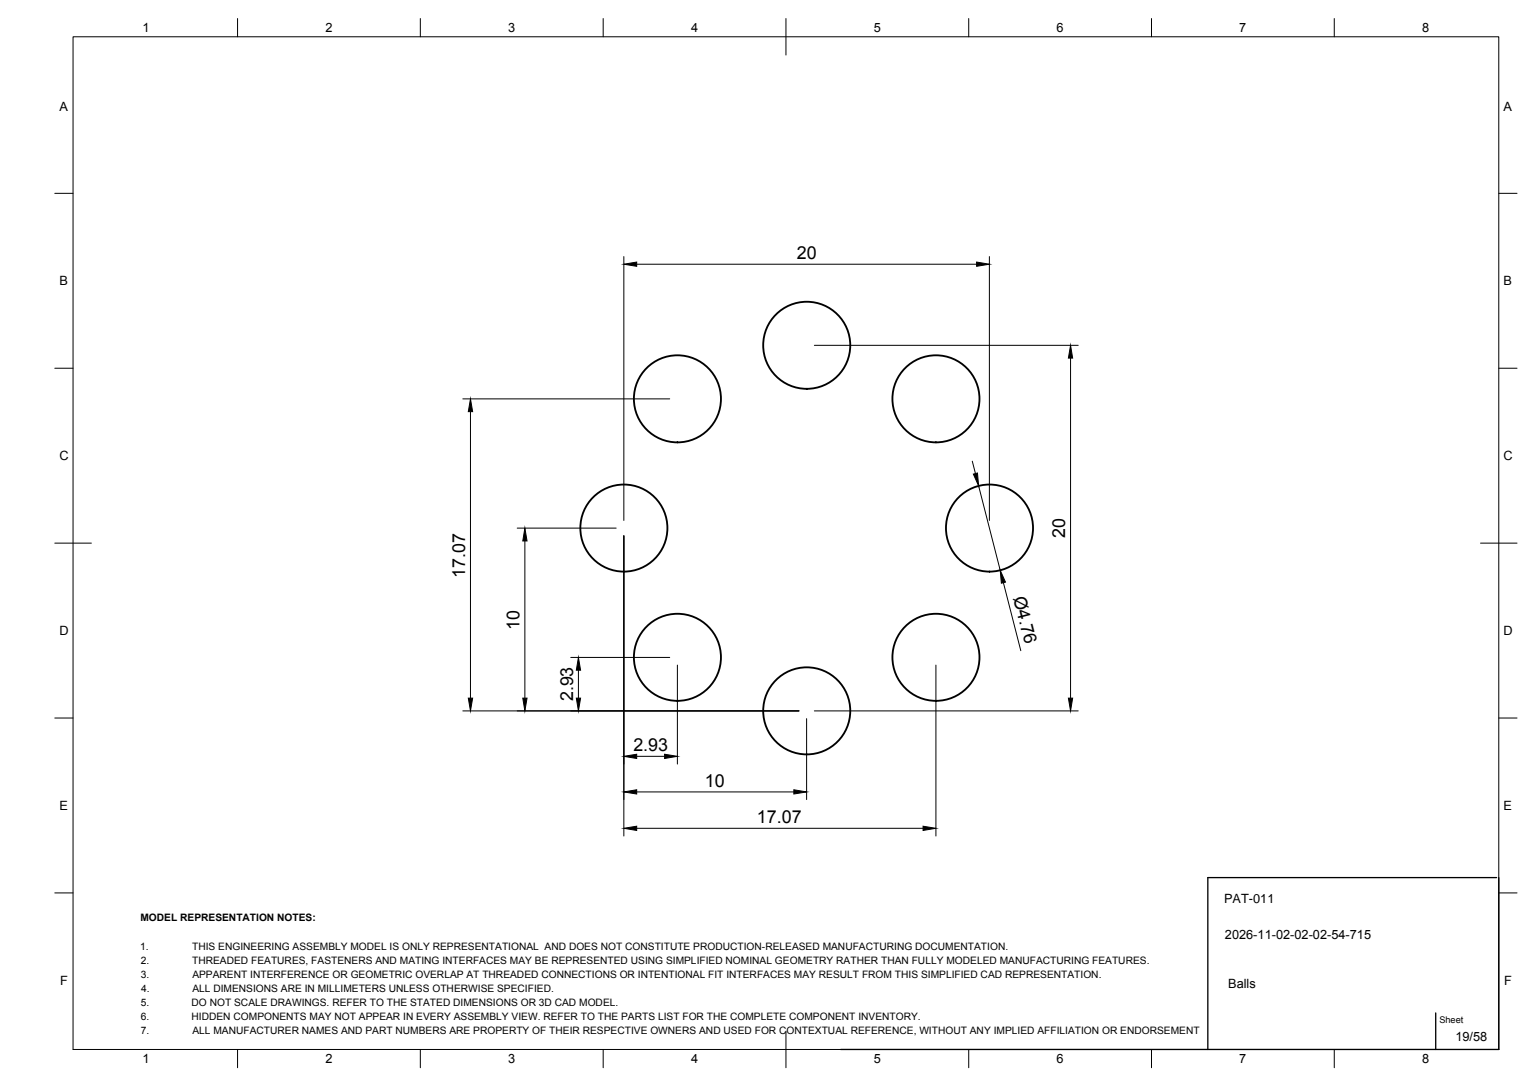
ISO-10303-21;
HEADER;
/* Generated by software containing ST-Developer
 * from STEP Tools, Inc. (www.steptools.com) 
 */

FILE_DESCRIPTION(
/* description */ ('Belt tension measurement rig'),
/* implementation_level */ '2;1');

FILE_NAME(
/* name */ 'Balls.step',
/* time_stamp */ '2026-10-28T03:24:44-07:00',
/* author */ (''),
/* organization */ (''),
/* preprocessor_version */ 'ST-DEVELOPER v20.2',
/* originating_system */ 'Autodesk Translation Framework v15.17.0.0',
/* authorisation */ '');

FILE_SCHEMA (('AUTOMOTIVE_DESIGN { 1 0 10303 214 3 1 1 }'));
ENDSEC;

DATA;
#10=MECHANICAL_DESIGN_GEOMETRIC_PRESENTATION_REPRESENTATION('',(#708,#709,#710,#711,#712,#713,#714,#715),#23587);
#437=SPHERICAL_SURFACE('',#13263,0.23815);
#438=SPHERICAL_SURFACE('',#13265,0.23815);
#439=SPHERICAL_SURFACE('',#13267,0.23815);
#440=SPHERICAL_SURFACE('',#13269,0.23815);
#441=SPHERICAL_SURFACE('',#13271,0.23815);
#442=SPHERICAL_SURFACE('',#13273,0.23815);
#443=SPHERICAL_SURFACE('',#13275,0.23815);
#444=SPHERICAL_SURFACE('',#13277,0.23815);
#598=SHAPE_REPRESENTATION_RELATIONSHIP('SRR','None',#23844,#653);
#653=ADVANCED_BREP_SHAPE_REPRESENTATION('',(#778,#779,#780,#781,#782,#783,
#784,#785),#23542);
#708=STYLED_ITEM('',(#24211),#778);
#709=STYLED_ITEM('',(#24211),#779);
#710=STYLED_ITEM('',(#24211),#780);
#711=STYLED_ITEM('',(#24211),#781);
#712=STYLED_ITEM('',(#24211),#782);
#713=STYLED_ITEM('',(#24211),#783);
#714=STYLED_ITEM('',(#24211),#784);
#715=STYLED_ITEM('',(#24211),#785);
#778=MANIFOLD_SOLID_BREP('Body1',#12213);
#779=MANIFOLD_SOLID_BREP('Body2',#12214);
#780=MANIFOLD_SOLID_BREP('Body3',#12215);
#781=MANIFOLD_SOLID_BREP('Body4',#12216);
#782=MANIFOLD_SOLID_BREP('Body5',#12217);
#783=MANIFOLD_SOLID_BREP('Body6',#12218);
#784=MANIFOLD_SOLID_BREP('Body7',#12219);
#785=MANIFOLD_SOLID_BREP('Body8',#12220);
#1545=FACE_OUTER_BOUND('',#2331,.T.);
#1546=FACE_OUTER_BOUND('',#2332,.T.);
#1547=FACE_OUTER_BOUND('',#2333,.T.);
#1548=FACE_OUTER_BOUND('',#2334,.T.);
#1549=FACE_OUTER_BOUND('',#2335,.T.);
#1550=FACE_OUTER_BOUND('',#2336,.T.);
#1551=FACE_OUTER_BOUND('',#2337,.T.);
#1552=FACE_OUTER_BOUND('',#2338,.T.);
#2331=EDGE_LOOP('',(#8748,#8749));
#2332=EDGE_LOOP('',(#8750,#8751));
#2333=EDGE_LOOP('',(#8752,#8753));
#2334=EDGE_LOOP('',(#8754,#8755));
#2335=EDGE_LOOP('',(#8756,#8757));
#2336=EDGE_LOOP('',(#8758,#8759));
#2337=EDGE_LOOP('',(#8760,#8761));
#2338=EDGE_LOOP('',(#8762,#8763));
#4644=CIRCLE('',#13264,0.23815);
#4645=CIRCLE('',#13266,0.23815);
#4646=CIRCLE('',#13268,0.23815);
#4647=CIRCLE('',#13270,0.23815);
#4648=CIRCLE('',#13272,0.23815);
#4649=CIRCLE('',#13274,0.23815);
#4650=CIRCLE('',#13276,0.23815);
#4651=CIRCLE('',#13278,0.23815);
#5504=VERTEX_POINT('',#19507);
#5505=VERTEX_POINT('',#19508);
#5506=VERTEX_POINT('',#19511);
#5507=VERTEX_POINT('',#19512);
#5508=VERTEX_POINT('',#19515);
#5509=VERTEX_POINT('',#19516);
#5510=VERTEX_POINT('',#19519);
#5511=VERTEX_POINT('',#19520);
#5512=VERTEX_POINT('',#19523);
#5513=VERTEX_POINT('',#19524);
#5514=VERTEX_POINT('',#19527);
#5515=VERTEX_POINT('',#19528);
#5516=VERTEX_POINT('',#19531);
#5517=VERTEX_POINT('',#19532);
#5518=VERTEX_POINT('',#19535);
#5519=VERTEX_POINT('',#19536);
#6733=EDGE_CURVE('',#5504,#5505,#4644,.T.);
#6734=EDGE_CURVE('',#5506,#5507,#4645,.T.);
#6735=EDGE_CURVE('',#5508,#5509,#4646,.T.);
#6736=EDGE_CURVE('',#5510,#5511,#4647,.T.);
#6737=EDGE_CURVE('',#5512,#5513,#4648,.T.);
#6738=EDGE_CURVE('',#5514,#5515,#4649,.T.);
#6739=EDGE_CURVE('',#5516,#5517,#4650,.T.);
#6740=EDGE_CURVE('',#5518,#5519,#4651,.T.);
#8748=ORIENTED_EDGE('',*,*,#6733,.T.);
#8749=ORIENTED_EDGE('',*,*,#6733,.F.);
#8750=ORIENTED_EDGE('',*,*,#6734,.T.);
#8751=ORIENTED_EDGE('',*,*,#6734,.F.);
#8752=ORIENTED_EDGE('',*,*,#6735,.T.);
#8753=ORIENTED_EDGE('',*,*,#6735,.F.);
#8754=ORIENTED_EDGE('',*,*,#6736,.T.);
#8755=ORIENTED_EDGE('',*,*,#6736,.F.);
#8756=ORIENTED_EDGE('',*,*,#6737,.T.);
#8757=ORIENTED_EDGE('',*,*,#6737,.F.);
#8758=ORIENTED_EDGE('',*,*,#6738,.T.);
#8759=ORIENTED_EDGE('',*,*,#6738,.F.);
#8760=ORIENTED_EDGE('',*,*,#6739,.T.);
#8761=ORIENTED_EDGE('',*,*,#6739,.F.);
#8762=ORIENTED_EDGE('',*,*,#6740,.T.);
#8763=ORIENTED_EDGE('',*,*,#6740,.F.);
#11686=ADVANCED_FACE('',(#1545),#437,.T.);
#11687=ADVANCED_FACE('',(#1546),#438,.T.);
#11688=ADVANCED_FACE('',(#1547),#439,.T.);
#11689=ADVANCED_FACE('',(#1548),#440,.T.);
#11690=ADVANCED_FACE('',(#1549),#441,.T.);
#11691=ADVANCED_FACE('',(#1550),#442,.T.);
#11692=ADVANCED_FACE('',(#1551),#443,.T.);
#11693=ADVANCED_FACE('',(#1552),#444,.T.);
#12213=CLOSED_SHELL('',(#11686));
#12214=CLOSED_SHELL('',(#11687));
#12215=CLOSED_SHELL('',(#11688));
#12216=CLOSED_SHELL('',(#11689));
#12217=CLOSED_SHELL('',(#11690));
#12218=CLOSED_SHELL('',(#11691));
#12219=CLOSED_SHELL('',(#11692));
#12220=CLOSED_SHELL('',(#11693));
#13262=AXIS2_PLACEMENT_3D('',#19505,#15516,#15517);
#13263=AXIS2_PLACEMENT_3D('',#19506,#15518,#15519);
#13264=AXIS2_PLACEMENT_3D('',#19509,#15520,#15521);
#13265=AXIS2_PLACEMENT_3D('',#19510,#15522,#15523);
#13266=AXIS2_PLACEMENT_3D('',#19513,#15524,#15525);
#13267=AXIS2_PLACEMENT_3D('',#19514,#15526,#15527);
#13268=AXIS2_PLACEMENT_3D('',#19517,#15528,#15529);
#13269=AXIS2_PLACEMENT_3D('',#19518,#15530,#15531);
#13270=AXIS2_PLACEMENT_3D('',#19521,#15532,#15533);
#13271=AXIS2_PLACEMENT_3D('',#19522,#15534,#15535);
#13272=AXIS2_PLACEMENT_3D('',#19525,#15536,#15537);
#13273=AXIS2_PLACEMENT_3D('',#19526,#15538,#15539);
#13274=AXIS2_PLACEMENT_3D('',#19529,#15540,#15541);
#13275=AXIS2_PLACEMENT_3D('',#19530,#15542,#15543);
#13276=AXIS2_PLACEMENT_3D('',#19533,#15544,#15545);
#13277=AXIS2_PLACEMENT_3D('',#19534,#15546,#15547);
#13278=AXIS2_PLACEMENT_3D('',#19537,#15548,#15549);
#15516=DIRECTION('axis',(0.,0.,1.));
#15517=DIRECTION('refdir',(1.,0.,0.));
#15518=DIRECTION('center_axis',(0.,0.,1.));
#15519=DIRECTION('ref_axis',(1.,0.,0.));
#15520=DIRECTION('center_axis',(1.22464679914735E-16,-1.,0.));
#15521=DIRECTION('ref_axis',(-1.,-1.22464679914735E-16,0.));
#15522=DIRECTION('center_axis',(0.707106781186548,0.,0.707106781186548));
#15523=DIRECTION('ref_axis',(0.707106781186548,0.,-0.707106781186548));
#15524=DIRECTION('center_axis',(8.65956056235494E-17,-1.,-8.65956056235493E-17));
#15525=DIRECTION('ref_axis',(-0.707106781186547,-1.22464679914735E-16,0.707106781186547));
#15526=DIRECTION('center_axis',(1.,0.,0.));
#15527=DIRECTION('ref_axis',(6.12323399573676E-17,0.,-1.));
#15528=DIRECTION('center_axis',(7.49879891330929E-33,-1.,-1.22464679914735E-16));
#15529=DIRECTION('ref_axis',(-6.12323399573676E-17,-1.22464679914735E-16,
1.));
#15530=DIRECTION('center_axis',(0.707106781186548,0.,-0.707106781186548));
#15531=DIRECTION('ref_axis',(-0.707106781186548,0.,-0.707106781186548));
#15532=DIRECTION('center_axis',(-8.65956056235493E-17,-1.,-8.65956056235494E-17));
#15533=DIRECTION('ref_axis',(0.707106781186547,-1.22464679914735E-16,0.707106781186547));
#15534=DIRECTION('center_axis',(0.,0.,-1.));
#15535=DIRECTION('ref_axis',(-1.,0.,-1.22464679914735E-16));
#15536=DIRECTION('center_axis',(-1.22464679914735E-16,-1.,-1.49975978266186E-32));
#15537=DIRECTION('ref_axis',(1.,-1.22464679914735E-16,1.22464679914735E-16));
#15538=DIRECTION('center_axis',(-0.707106781186547,0.,-0.707106781186548));
#15539=DIRECTION('ref_axis',(-0.707106781186548,0.,0.707106781186547));
#15540=DIRECTION('center_axis',(-8.65956056235493E-17,-1.,8.65956056235493E-17));
#15541=DIRECTION('ref_axis',(0.707106781186548,-1.22464679914735E-16,-0.707106781186547));
#15542=DIRECTION('center_axis',(-1.,0.,0.));
#15543=DIRECTION('ref_axis',(-1.83697019872103E-16,0.,1.));
#15544=DIRECTION('center_axis',(-2.24963967399279E-32,-1.,1.22464679914735E-16));
#15545=DIRECTION('ref_axis',(1.83697019872103E-16,-1.22464679914735E-16,
-1.));
#15546=DIRECTION('center_axis',(-0.707106781186548,0.,0.707106781186548));
#15547=DIRECTION('ref_axis',(0.707106781186547,0.,0.707106781186548));
#15548=DIRECTION('center_axis',(8.65956056235493E-17,-1.,8.65956056235493E-17));
#15549=DIRECTION('ref_axis',(-0.707106781186547,-1.22464679914735E-16,-0.707106781186548));
#19505=CARTESIAN_POINT('',(0.,0.,0.));
#19506=CARTESIAN_POINT('Origin',(1.,0.,0.));
#19507=CARTESIAN_POINT('',(1.,-1.78583896120461E-33,0.23815));
#19508=CARTESIAN_POINT('',(1.,-1.78583896120461E-33,-0.23815));
#19509=CARTESIAN_POINT('Origin',(1.,0.,0.));
#19510=CARTESIAN_POINT('Origin',(0.707106781186548,0.,-0.707106781186547));
#19511=CARTESIAN_POINT('',(0.875504261126124,-1.78583896120461E-33,-0.538709301246971));
#19512=CARTESIAN_POINT('',(0.538709301246971,-1.78583896120461E-33,-0.875504261126124));
#19513=CARTESIAN_POINT('Origin',(0.707106781186548,0.,-0.707106781186547));
#19514=CARTESIAN_POINT('Origin',(6.12323399573677E-17,0.,-1.));
#19515=CARTESIAN_POINT('',(0.23815,-1.78583896120461E-33,-1.));
#19516=CARTESIAN_POINT('',(-0.23815,-1.78583896120461E-33,-1.));
#19517=CARTESIAN_POINT('Origin',(6.12323399573677E-17,0.,-1.));
#19518=CARTESIAN_POINT('Origin',(-0.707106781186547,0.,-0.707106781186548));
#19519=CARTESIAN_POINT('',(-0.538709301246971,-1.78583896120461E-33,-0.875504261126124));
#19520=CARTESIAN_POINT('',(-0.875504261126124,-1.78583896120461E-33,-0.538709301246971));
#19521=CARTESIAN_POINT('Origin',(-0.707106781186547,0.,-0.707106781186548));
#19522=CARTESIAN_POINT('Origin',(-1.,0.,-1.22464679914735E-16));
#19523=CARTESIAN_POINT('',(-1.,-1.78583896120461E-33,-0.23815));
#19524=CARTESIAN_POINT('',(-1.,-1.78583896120461E-33,0.23815));
#19525=CARTESIAN_POINT('Origin',(-1.,0.,-1.22464679914735E-16));
#19526=CARTESIAN_POINT('Origin',(-0.707106781186548,0.,0.707106781186547));
#19527=CARTESIAN_POINT('',(-0.875504261126124,-7.94881478324376E-33,0.538709301246971));
#19528=CARTESIAN_POINT('',(-0.538709301246971,4.37713686083455E-33,0.875504261126124));
#19529=CARTESIAN_POINT('Origin',(-0.707106781186548,0.,0.707106781186547));
#19530=CARTESIAN_POINT('Origin',(-1.83697019872103E-16,0.,1.));
#19531=CARTESIAN_POINT('',(-0.23815,-1.78583896120461E-33,1.));
#19532=CARTESIAN_POINT('',(0.23815,-1.78583896120461E-33,1.));
#19533=CARTESIAN_POINT('Origin',(-1.83697019872103E-16,0.,1.));
#19534=CARTESIAN_POINT('Origin',(0.707106781186547,0.,0.707106781186548));
#19535=CARTESIAN_POINT('',(0.538709301246971,-4.86732687222419E-33,0.875504261126124));
#19536=CARTESIAN_POINT('',(0.875504261126124,1.29564894981497E-33,0.538709301246971));
#19537=CARTESIAN_POINT('Origin',(0.707106781186547,0.,0.707106781186548));
#23477=UNCERTAINTY_MEASURE_WITH_UNIT(LENGTH_MEASURE(0.001),#23588,
'DISTANCE_ACCURACY_VALUE',
'Maximum model space distance between geometric entities at asserted c
onnectivities');
#23522=UNCERTAINTY_MEASURE_WITH_UNIT(LENGTH_MEASURE(0.001),#23588,
'DISTANCE_ACCURACY_VALUE',
'Maximum model space distance between geometric entities at asserted c
onnectivities');
#23542=(
GEOMETRIC_REPRESENTATION_CONTEXT(3)
GLOBAL_UNCERTAINTY_ASSIGNED_CONTEXT((#23477))
GLOBAL_UNIT_ASSIGNED_CONTEXT((#23588,#23590,#23591))
REPRESENTATION_CONTEXT('','3D')
);
#23587=(
GEOMETRIC_REPRESENTATION_CONTEXT(3)
GLOBAL_UNCERTAINTY_ASSIGNED_CONTEXT((#23522))
GLOBAL_UNIT_ASSIGNED_CONTEXT((#23588,#23590,#23591))
REPRESENTATION_CONTEXT('','3D')
);
#23588=(
LENGTH_UNIT()
NAMED_UNIT(*)
SI_UNIT(.CENTI.,.METRE.)
);
#23590=(
NAMED_UNIT(*)
PLANE_ANGLE_UNIT()
SI_UNIT($,.RADIAN.)
);
#23591=(
NAMED_UNIT(*)
SI_UNIT($,.STERADIAN.)
SOLID_ANGLE_UNIT()
);
#23611=SHAPE_DEFINITION_REPRESENTATION(#23675,#23844);
#23675=PRODUCT_DEFINITION_SHAPE('',$,#23909);
#23844=SHAPE_REPRESENTATION('',(#13262),#23542);
#23889=PRODUCT_DEFINITION_CONTEXT('part definition',#24083,'design');
#23909=PRODUCT_DEFINITION('Balls','Balls',#23973,#23889);
#23973=PRODUCT_DEFINITION_FORMATION('',$,#24104);
#24083=APPLICATION_CONTEXT(
'Core Data for Automotive Mechanical Design Process');
#24084=PRODUCT_CONTEXT('part definition',#24083,'mechanical');
#24104=PRODUCT('Balls','Balls','Balls',(#24084));
#24205=COLOUR_RGB('Grey',0.48,0.52,0.57);
#24206=FILL_AREA_STYLE_COLOUR('',#24205);
#24207=FILL_AREA_STYLE('',(#24206));
#24208=SURFACE_STYLE_FILL_AREA(#24207);
#24209=SURFACE_SIDE_STYLE('',(#24208));
#24210=SURFACE_STYLE_USAGE(.BOTH.,#24209);
#24211=PRESENTATION_STYLE_ASSIGNMENT((#24210));
ENDSEC;
END-ISO-10303-21;
